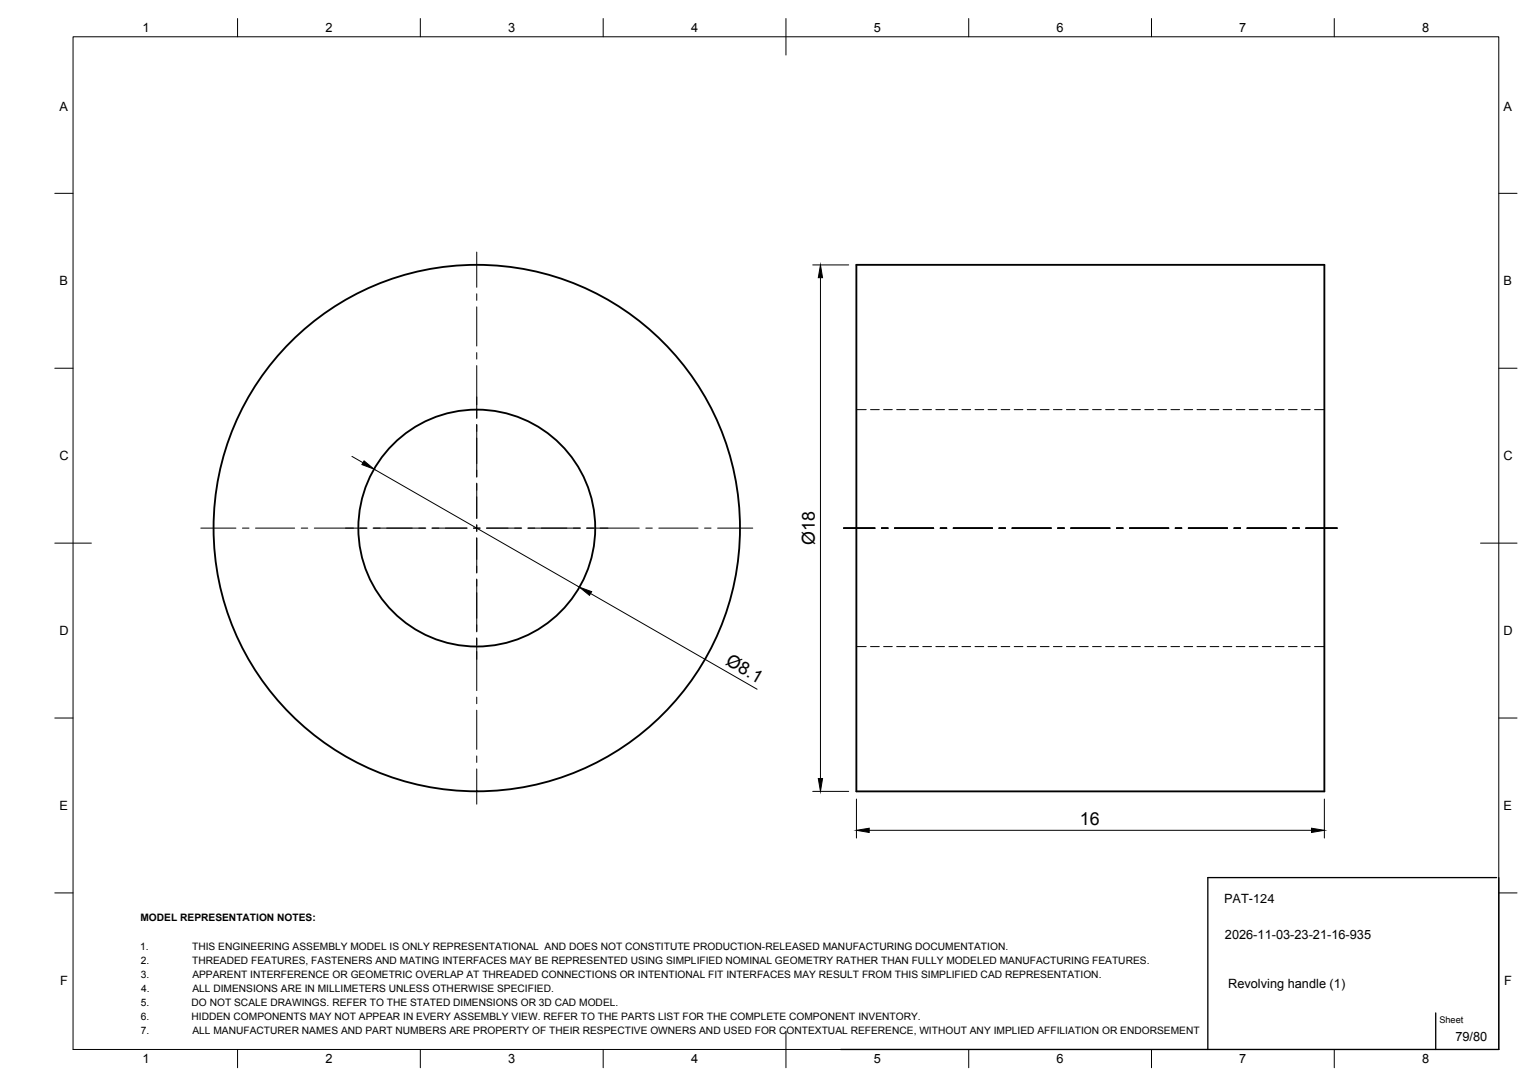
ISO-10303-21;
HEADER;
/* Generated by software containing ST-Developer
 * from STEP Tools, Inc. (www.steptools.com) 
 */

FILE_DESCRIPTION(
/* description */ ('XY cross-slide table'),
/* implementation_level */ '2;1');

FILE_NAME(
/* name */ 'Revolving handle (1).step',
/* time_stamp */ '2026-10-28T03:22:46-07:00',
/* author */ (''),
/* organization */ (''),
/* preprocessor_version */ 'ST-DEVELOPER v20.2',
/* originating_system */ 'Autodesk Translation Framework v15.17.0.0',
/* authorisation */ '');

FILE_SCHEMA (('AUTOMOTIVE_DESIGN { 1 0 10303 214 3 1 1 }'));
ENDSEC;

DATA;
#10=MECHANICAL_DESIGN_GEOMETRIC_PRESENTATION_REPRESENTATION('',(#1778),#62984);
#1582=SHAPE_REPRESENTATION_RELATIONSHIP('SRR','None',#63442,#1665);
#1665=ADVANCED_BREP_SHAPE_REPRESENTATION('',(#1883),#62979);
#1778=STYLED_ITEM('',(#63905),#1883);
#1883=MANIFOLD_SOLID_BREP('Body1',#23080);
#2290=FACE_BOUND('',#5856,.T.);
#2291=FACE_BOUND('',#5858,.T.);
#2835=PLANE('',#26345);
#2836=PLANE('',#26346);
#4136=FACE_OUTER_BOUND('',#5853,.T.);
#4137=FACE_OUTER_BOUND('',#5854,.T.);
#4138=FACE_OUTER_BOUND('',#5855,.T.);
#4139=FACE_OUTER_BOUND('',#5857,.T.);
#5853=EDGE_LOOP('',(#20854,#20855,#20856,#20857));
#5854=EDGE_LOOP('',(#20858,#20859,#20860,#20861));
#5855=EDGE_LOOP('',(#20862));
#5856=EDGE_LOOP('',(#20863));
#5857=EDGE_LOOP('',(#20864));
#5858=EDGE_LOOP('',(#20865));
#7320=LINE('',#62536,#8807);
#7321=LINE('',#62542,#8808);
#8807=VECTOR('',#32557,0.405);
#8808=VECTOR('',#32564,0.9);
#9753=CIRCLE('',#26340,0.405);
#9754=CIRCLE('',#26341,0.405);
#9755=CIRCLE('',#26343,0.9);
#9756=CIRCLE('',#26344,0.9);
#11776=VERTEX_POINT('',#62533);
#11777=VERTEX_POINT('',#62535);
#11778=VERTEX_POINT('',#62539);
#11779=VERTEX_POINT('',#62541);
#14811=EDGE_CURVE('',#11776,#11776,#9753,.T.);
#14812=EDGE_CURVE('',#11776,#11777,#7320,.T.);
#14813=EDGE_CURVE('',#11777,#11777,#9754,.T.);
#14814=EDGE_CURVE('',#11778,#11778,#9755,.T.);
#14815=EDGE_CURVE('',#11778,#11779,#7321,.T.);
#14816=EDGE_CURVE('',#11779,#11779,#9756,.T.);
#20854=ORIENTED_EDGE('',*,*,#14811,.F.);
#20855=ORIENTED_EDGE('',*,*,#14812,.T.);
#20856=ORIENTED_EDGE('',*,*,#14813,.T.);
#20857=ORIENTED_EDGE('',*,*,#14812,.F.);
#20858=ORIENTED_EDGE('',*,*,#14814,.F.);
#20859=ORIENTED_EDGE('',*,*,#14815,.T.);
#20860=ORIENTED_EDGE('',*,*,#14816,.T.);
#20861=ORIENTED_EDGE('',*,*,#14815,.F.);
#20862=ORIENTED_EDGE('',*,*,#14814,.T.);
#20863=ORIENTED_EDGE('',*,*,#14811,.T.);
#20864=ORIENTED_EDGE('',*,*,#14816,.F.);
#20865=ORIENTED_EDGE('',*,*,#14813,.F.);
#21643=CYLINDRICAL_SURFACE('',#26339,0.405);
#21644=CYLINDRICAL_SURFACE('',#26342,0.9);
#22917=ADVANCED_FACE('',(#4136),#21643,.F.);
#22918=ADVANCED_FACE('',(#4137),#21644,.T.);
#22919=ADVANCED_FACE('',(#4138,#2290),#2835,.T.);
#22920=ADVANCED_FACE('',(#4139,#2291),#2836,.F.);
#23080=CLOSED_SHELL('',(#22917,#22918,#22919,#22920));
#26338=AXIS2_PLACEMENT_3D('',#62531,#32551,#32552);
#26339=AXIS2_PLACEMENT_3D('',#62532,#32553,#32554);
#26340=AXIS2_PLACEMENT_3D('',#62534,#32555,#32556);
#26341=AXIS2_PLACEMENT_3D('',#62537,#32558,#32559);
#26342=AXIS2_PLACEMENT_3D('',#62538,#32560,#32561);
#26343=AXIS2_PLACEMENT_3D('',#62540,#32562,#32563);
#26344=AXIS2_PLACEMENT_3D('',#62543,#32565,#32566);
#26345=AXIS2_PLACEMENT_3D('',#62544,#32567,#32568);
#26346=AXIS2_PLACEMENT_3D('',#62545,#32569,#32570);
#32551=DIRECTION('axis',(0.,0.,1.));
#32552=DIRECTION('refdir',(1.,0.,0.));
#32553=DIRECTION('center_axis',(1.,0.,0.));
#32554=DIRECTION('ref_axis',(0.,0.,-1.));
#32555=DIRECTION('center_axis',(-1.,0.,0.));
#32556=DIRECTION('ref_axis',(0.,0.,-1.));
#32557=DIRECTION('',(-1.,0.,0.));
#32558=DIRECTION('center_axis',(-1.,0.,0.));
#32559=DIRECTION('ref_axis',(0.,0.,-1.));
#32560=DIRECTION('center_axis',(1.,0.,0.));
#32561=DIRECTION('ref_axis',(0.,0.,-1.));
#32562=DIRECTION('center_axis',(1.,0.,0.));
#32563=DIRECTION('ref_axis',(0.,0.,-1.));
#32564=DIRECTION('',(-1.,0.,0.));
#32565=DIRECTION('center_axis',(1.,0.,0.));
#32566=DIRECTION('ref_axis',(0.,0.,-1.));
#32567=DIRECTION('center_axis',(1.,0.,0.));
#32568=DIRECTION('ref_axis',(0.,0.,-1.));
#32569=DIRECTION('center_axis',(1.,0.,0.));
#32570=DIRECTION('ref_axis',(0.,0.,-1.));
#62531=CARTESIAN_POINT('',(0.,0.,0.));
#62532=CARTESIAN_POINT('Origin',(29.4,0.,6.5));
#62533=CARTESIAN_POINT('',(31.,-4.95981953654678E-17,6.905));
#62534=CARTESIAN_POINT('Origin',(31.,0.,6.5));
#62535=CARTESIAN_POINT('',(29.4,-4.95981953654678E-17,6.905));
#62536=CARTESIAN_POINT('',(29.4,-4.95981953654678E-17,6.905));
#62537=CARTESIAN_POINT('Origin',(29.4,0.,6.5));
#62538=CARTESIAN_POINT('Origin',(29.4,0.,6.5));
#62539=CARTESIAN_POINT('',(31.,-1.10218211923262E-16,7.4));
#62540=CARTESIAN_POINT('Origin',(31.,0.,6.5));
#62541=CARTESIAN_POINT('',(29.4,-1.10218211923262E-16,7.4));
#62542=CARTESIAN_POINT('',(29.4,-1.10218211923262E-16,7.4));
#62543=CARTESIAN_POINT('Origin',(29.4,0.,6.5));
#62544=CARTESIAN_POINT('Origin',(31.,0.,6.5));
#62545=CARTESIAN_POINT('Origin',(29.4,0.,6.5));
#62880=UNCERTAINTY_MEASURE_WITH_UNIT(LENGTH_MEASURE(0.001),#62985,
'DISTANCE_ACCURACY_VALUE',
'Maximum model space distance between geometric entities at asserted c
onnectivities');
#62885=UNCERTAINTY_MEASURE_WITH_UNIT(LENGTH_MEASURE(0.001),#62985,
'DISTANCE_ACCURACY_VALUE',
'Maximum model space distance between geometric entities at asserted c
onnectivities');
#62979=(
GEOMETRIC_REPRESENTATION_CONTEXT(3)
GLOBAL_UNCERTAINTY_ASSIGNED_CONTEXT((#62880))
GLOBAL_UNIT_ASSIGNED_CONTEXT((#62985,#62987,#62988))
REPRESENTATION_CONTEXT('','3D')
);
#62984=(
GEOMETRIC_REPRESENTATION_CONTEXT(3)
GLOBAL_UNCERTAINTY_ASSIGNED_CONTEXT((#62885))
GLOBAL_UNIT_ASSIGNED_CONTEXT((#62985,#62987,#62988))
REPRESENTATION_CONTEXT('','3D')
);
#62985=(
LENGTH_UNIT()
NAMED_UNIT(*)
SI_UNIT(.CENTI.,.METRE.)
);
#62987=(
NAMED_UNIT(*)
PLANE_ANGLE_UNIT()
SI_UNIT($,.RADIAN.)
);
#62988=(
NAMED_UNIT(*)
SI_UNIT($,.STERADIAN.)
SOLID_ANGLE_UNIT()
);
#63082=SHAPE_DEFINITION_REPRESENTATION(#63293,#63442);
#63293=PRODUCT_DEFINITION_SHAPE('',$,#63541);
#63442=SHAPE_REPRESENTATION('',(#26338),#62979);
#63447=PRODUCT_DEFINITION_CONTEXT('part definition',#63743,'design');
#63541=PRODUCT_DEFINITION('Revolving handle (1)','Revolving handle (1)',#63639,
#63447);
#63639=PRODUCT_DEFINITION_FORMATION('',$,#63838);
#63743=APPLICATION_CONTEXT(
'Core Data for Automotive Mechanical Design Process');
#63744=PRODUCT_CONTEXT('part definition',#63743,'mechanical');
#63838=PRODUCT('Revolving handle (1)','Revolving handle (1)',
'Revolving handle (1)',(#63744));
#63899=COLOUR_RGB('Sky Blue',0.24,0.69,0.87);
#63900=FILL_AREA_STYLE_COLOUR('',#63899);
#63901=FILL_AREA_STYLE('',(#63900));
#63902=SURFACE_STYLE_FILL_AREA(#63901);
#63903=SURFACE_SIDE_STYLE('',(#63902));
#63904=SURFACE_STYLE_USAGE(.BOTH.,#63903);
#63905=PRESENTATION_STYLE_ASSIGNMENT((#63904));
ENDSEC;
END-ISO-10303-21;
